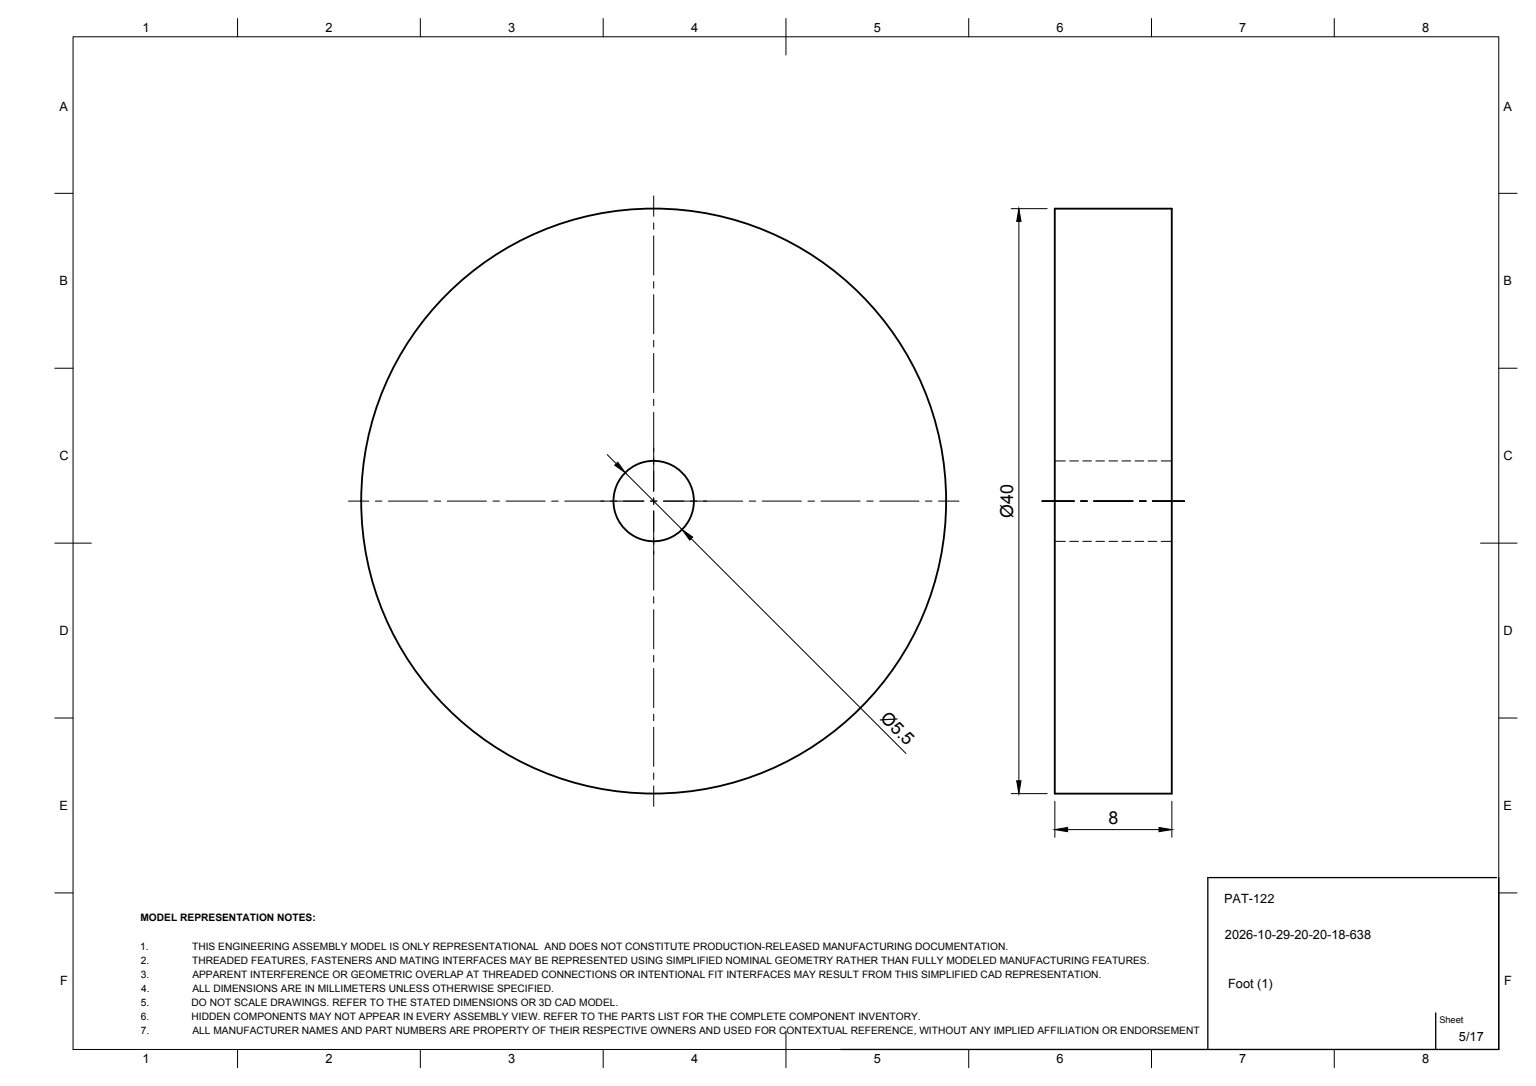
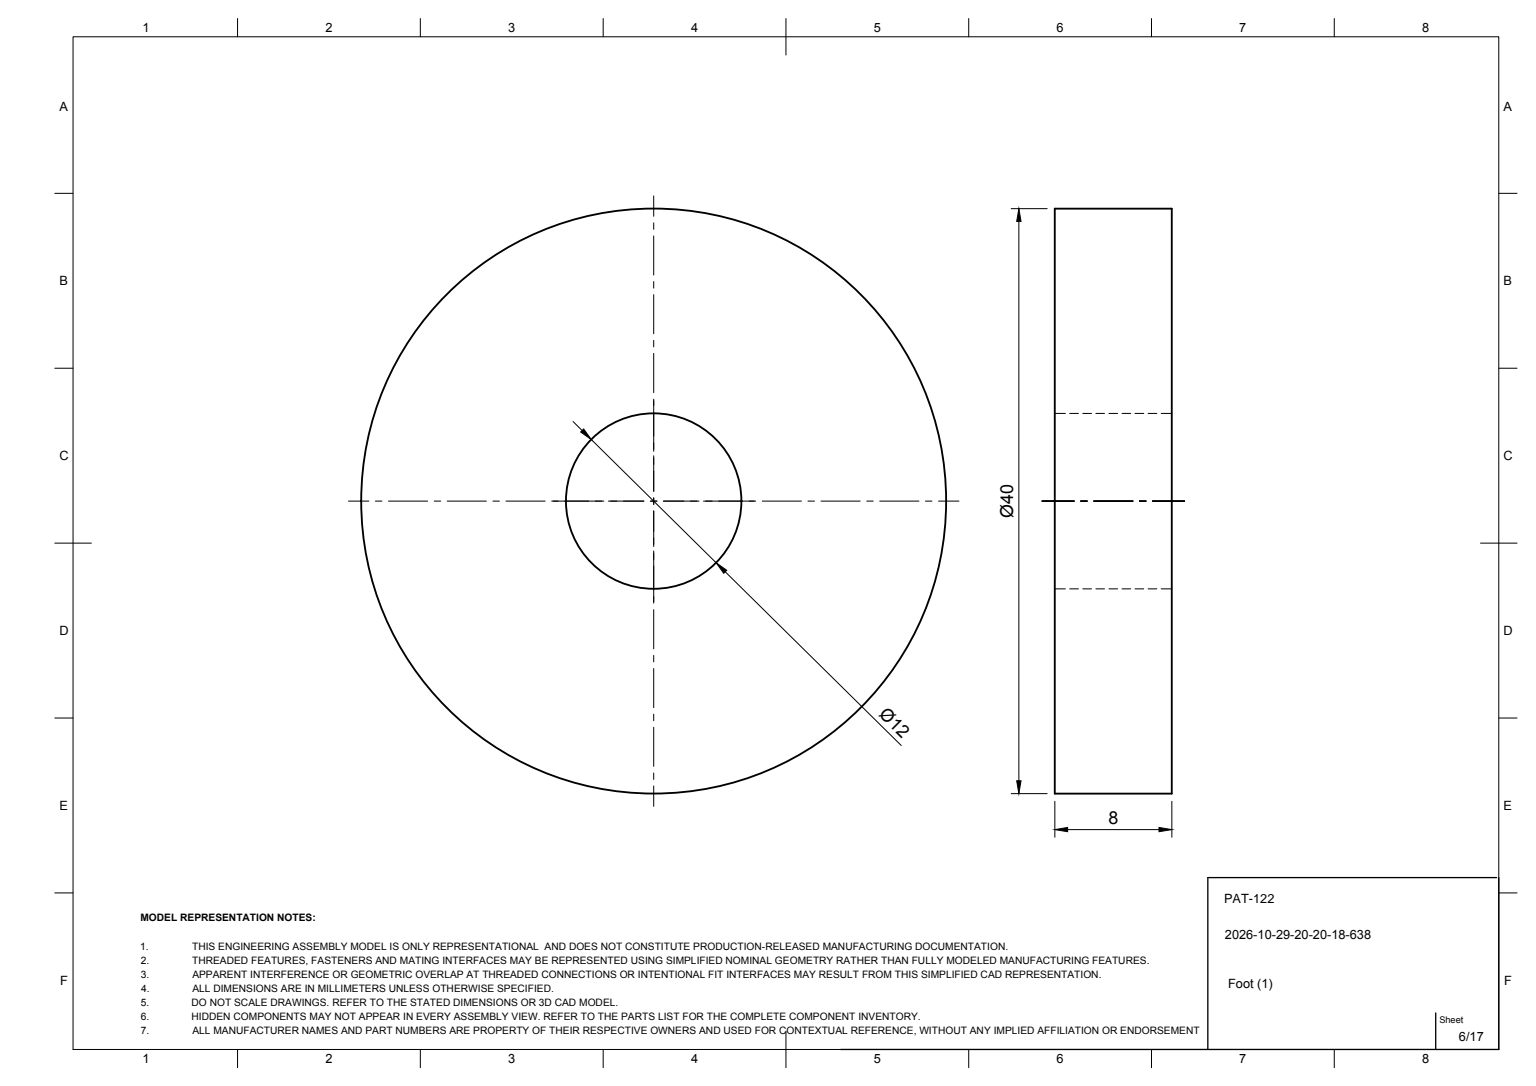
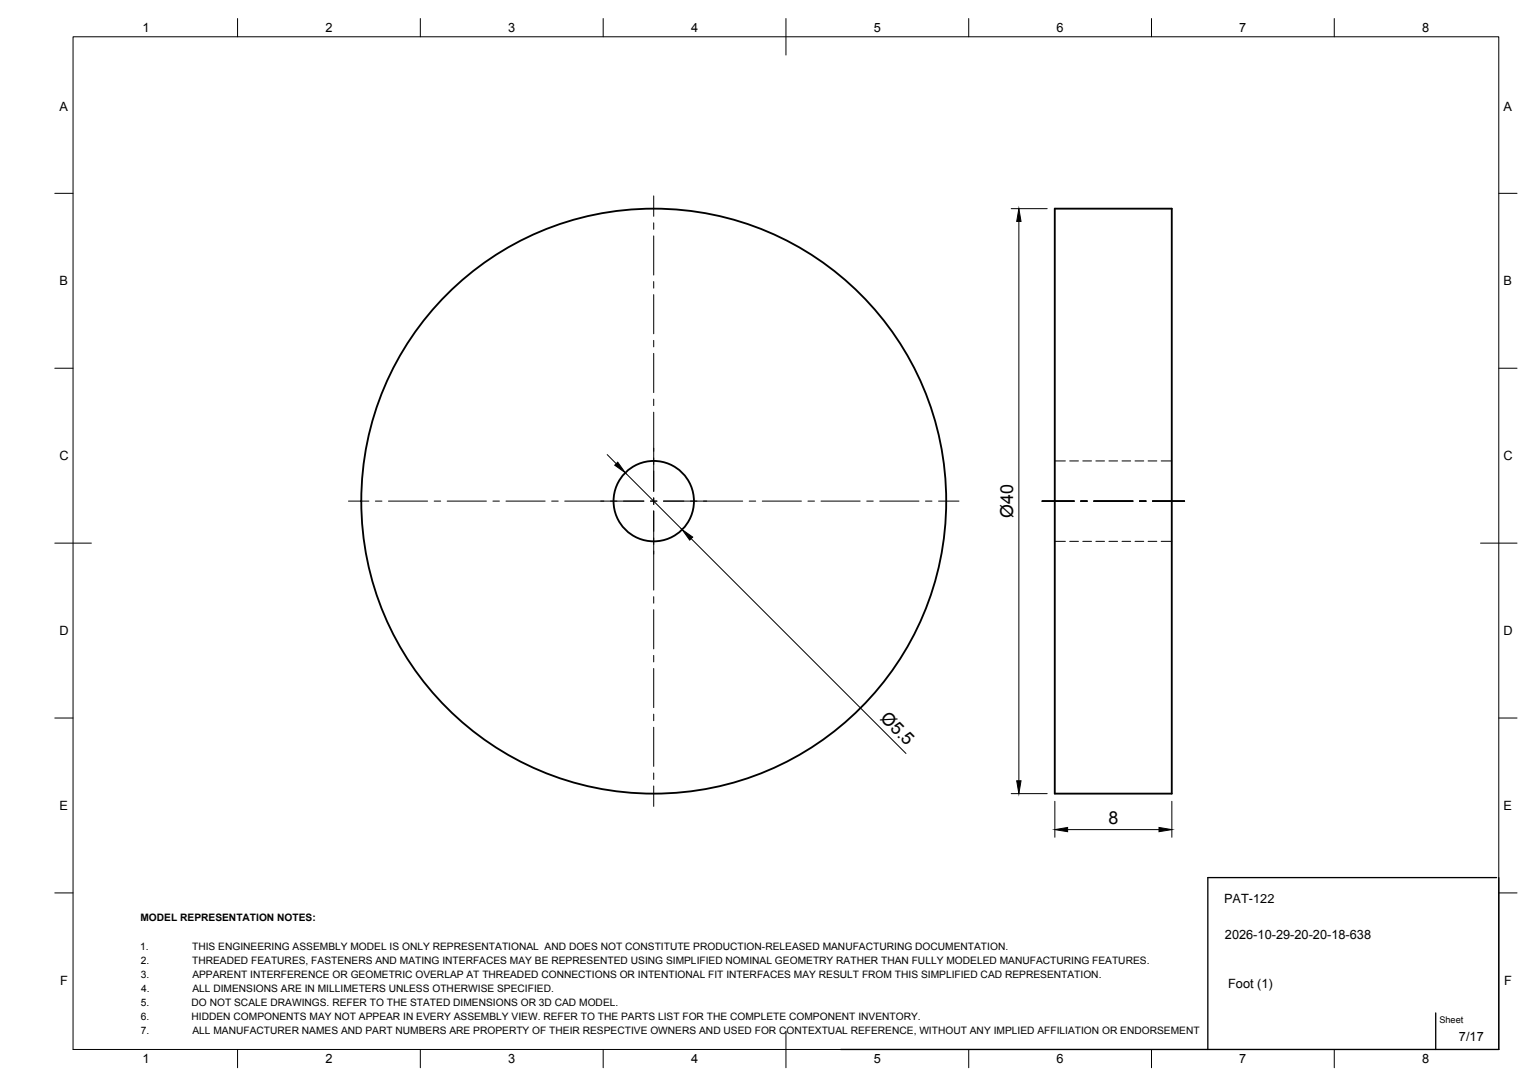
ISO-10303-21;
HEADER;
/* Generated by software containing ST-Developer
 * from STEP Tools, Inc. (www.steptools.com) 
 */

FILE_DESCRIPTION(
/* description */ ('PAT-122'),
/* implementation_level */ '2;1');

FILE_NAME(
/* name */ 'Foot (1).step',
/* time_stamp */ '2026-10-29T20:20:12-07:00',
/* author */ (''),
/* organization */ (''),
/* preprocessor_version */ 'ST-DEVELOPER v20.2',
/* originating_system */ 'Autodesk Translation Framework v15.17.0.0',
/* authorisation */ '');

FILE_SCHEMA (('AUTOMOTIVE_DESIGN { 1 0 10303 214 3 1 1 }'));
ENDSEC;

DATA;
#10=MECHANICAL_DESIGN_GEOMETRIC_PRESENTATION_REPRESENTATION('',(#493),#10019);
#449=SHAPE_REPRESENTATION_RELATIONSHIP('SRR','None',#10170,#471);
#471=ADVANCED_BREP_SHAPE_REPRESENTATION('',(#515),#9999);
#493=STYLED_ITEM('',(#10362),#515);
#515=MANIFOLD_SOLID_BREP('Body1',#5615);
#535=FACE_BOUND('',#1132,.T.);
#536=FACE_BOUND('',#1134,.T.);
#613=PLANE('',#5908);
#614=PLANE('',#5909);
#833=FACE_OUTER_BOUND('',#1129,.T.);
#834=FACE_OUTER_BOUND('',#1130,.T.);
#835=FACE_OUTER_BOUND('',#1131,.T.);
#836=FACE_OUTER_BOUND('',#1133,.T.);
#1129=EDGE_LOOP('',(#3889,#3890,#3891,#3892));
#1130=EDGE_LOOP('',(#3893,#3894,#3895,#3896));
#1131=EDGE_LOOP('',(#3897));
#1132=EDGE_LOOP('',(#3898));
#1133=EDGE_LOOP('',(#3899));
#1134=EDGE_LOOP('',(#3900));
#1491=LINE('',#8094,#2035);
#1492=LINE('',#8100,#2036);
#2035=VECTOR('',#6474,0.274999999999999);
#2036=VECTOR('',#6481,2.);
#2583=CIRCLE('',#5903,0.274999999999999);
#2584=CIRCLE('',#5904,0.274999999999999);
#2585=CIRCLE('',#5906,2.);
#2586=CIRCLE('',#5907,2.);
#2713=VERTEX_POINT('',#8091);
#2714=VERTEX_POINT('',#8093);
#2715=VERTEX_POINT('',#8097);
#2716=VERTEX_POINT('',#8099);
#3179=EDGE_CURVE('',#2713,#2713,#2583,.T.);
#3180=EDGE_CURVE('',#2713,#2714,#1491,.T.);
#3181=EDGE_CURVE('',#2714,#2714,#2584,.T.);
#3182=EDGE_CURVE('',#2715,#2715,#2585,.T.);
#3183=EDGE_CURVE('',#2715,#2716,#1492,.T.);
#3184=EDGE_CURVE('',#2716,#2716,#2586,.T.);
#3889=ORIENTED_EDGE('',*,*,#3179,.F.);
#3890=ORIENTED_EDGE('',*,*,#3180,.T.);
#3891=ORIENTED_EDGE('',*,*,#3181,.T.);
#3892=ORIENTED_EDGE('',*,*,#3180,.F.);
#3893=ORIENTED_EDGE('',*,*,#3182,.F.);
#3894=ORIENTED_EDGE('',*,*,#3183,.T.);
#3895=ORIENTED_EDGE('',*,*,#3184,.T.);
#3896=ORIENTED_EDGE('',*,*,#3183,.F.);
#3897=ORIENTED_EDGE('',*,*,#3182,.T.);
#3898=ORIENTED_EDGE('',*,*,#3179,.T.);
#3899=ORIENTED_EDGE('',*,*,#3184,.F.);
#3900=ORIENTED_EDGE('',*,*,#3181,.F.);
#5265=CYLINDRICAL_SURFACE('',#5902,0.274999999999999);
#5266=CYLINDRICAL_SURFACE('',#5905,2.);
#5329=ADVANCED_FACE('',(#833),#5265,.F.);
#5330=ADVANCED_FACE('',(#834),#5266,.T.);
#5331=ADVANCED_FACE('',(#835,#535),#613,.T.);
#5332=ADVANCED_FACE('',(#836,#536),#614,.F.);
#5615=CLOSED_SHELL('',(#5329,#5330,#5331,#5332));
#5901=AXIS2_PLACEMENT_3D('',#8089,#6468,#6469);
#5902=AXIS2_PLACEMENT_3D('',#8090,#6470,#6471);
#5903=AXIS2_PLACEMENT_3D('',#8092,#6472,#6473);
#5904=AXIS2_PLACEMENT_3D('',#8095,#6475,#6476);
#5905=AXIS2_PLACEMENT_3D('',#8096,#6477,#6478);
#5906=AXIS2_PLACEMENT_3D('',#8098,#6479,#6480);
#5907=AXIS2_PLACEMENT_3D('',#8101,#6482,#6483);
#5908=AXIS2_PLACEMENT_3D('',#8102,#6484,#6485);
#5909=AXIS2_PLACEMENT_3D('',#8103,#6486,#6487);
#6468=DIRECTION('axis',(0.,0.,1.));
#6469=DIRECTION('refdir',(1.,0.,0.));
#6470=DIRECTION('center_axis',(0.,0.,1.));
#6471=DIRECTION('ref_axis',(1.,0.,0.));
#6472=DIRECTION('center_axis',(0.,0.,-1.));
#6473=DIRECTION('ref_axis',(1.,0.,0.));
#6474=DIRECTION('',(0.,0.,-1.));
#6475=DIRECTION('center_axis',(0.,0.,-1.));
#6476=DIRECTION('ref_axis',(1.,0.,0.));
#6477=DIRECTION('center_axis',(0.,0.,1.));
#6478=DIRECTION('ref_axis',(1.,0.,0.));
#6479=DIRECTION('center_axis',(0.,0.,1.));
#6480=DIRECTION('ref_axis',(1.,0.,0.));
#6481=DIRECTION('',(0.,0.,-1.));
#6482=DIRECTION('center_axis',(0.,0.,1.));
#6483=DIRECTION('ref_axis',(1.,0.,0.));
#6484=DIRECTION('center_axis',(0.,0.,1.));
#6485=DIRECTION('ref_axis',(1.,0.,0.));
#6486=DIRECTION('center_axis',(0.,0.,1.));
#6487=DIRECTION('ref_axis',(1.,0.,0.));
#8089=CARTESIAN_POINT('',(0.,0.,0.));
#8090=CARTESIAN_POINT('Origin',(-19.,19.,-0.8));
#8091=CARTESIAN_POINT('',(-19.275,19.,0.));
#8092=CARTESIAN_POINT('Origin',(-19.,19.,0.));
#8093=CARTESIAN_POINT('',(-19.275,19.,-0.8));
#8094=CARTESIAN_POINT('',(-19.275,19.,-0.8));
#8095=CARTESIAN_POINT('Origin',(-19.,19.,-0.8));
#8096=CARTESIAN_POINT('Origin',(-19.,19.,-0.8));
#8097=CARTESIAN_POINT('',(-21.,19.,0.));
#8098=CARTESIAN_POINT('Origin',(-19.,19.,0.));
#8099=CARTESIAN_POINT('',(-21.,19.,-0.8));
#8100=CARTESIAN_POINT('',(-21.,19.,-0.8));
#8101=CARTESIAN_POINT('Origin',(-19.,19.,-0.8));
#8102=CARTESIAN_POINT('Origin',(-19.,19.,0.));
#8103=CARTESIAN_POINT('Origin',(-19.,19.,-0.8));
#9975=UNCERTAINTY_MEASURE_WITH_UNIT(LENGTH_MEASURE(0.001),#10020,
'DISTANCE_ACCURACY_VALUE',
'Maximum model space distance between geometric entities at asserted c
onnectivities');
#9995=UNCERTAINTY_MEASURE_WITH_UNIT(LENGTH_MEASURE(0.001),#10020,
'DISTANCE_ACCURACY_VALUE',
'Maximum model space distance between geometric entities at asserted c
onnectivities');
#9999=(
GEOMETRIC_REPRESENTATION_CONTEXT(3)
GLOBAL_UNCERTAINTY_ASSIGNED_CONTEXT((#9975))
GLOBAL_UNIT_ASSIGNED_CONTEXT((#10020,#10022,#10023))
REPRESENTATION_CONTEXT('','3D')
);
#10019=(
GEOMETRIC_REPRESENTATION_CONTEXT(3)
GLOBAL_UNCERTAINTY_ASSIGNED_CONTEXT((#9995))
GLOBAL_UNIT_ASSIGNED_CONTEXT((#10020,#10022,#10023))
REPRESENTATION_CONTEXT('','3D')
);
#10020=(
LENGTH_UNIT()
NAMED_UNIT(*)
SI_UNIT(.CENTI.,.METRE.)
);
#10022=(
NAMED_UNIT(*)
PLANE_ANGLE_UNIT()
SI_UNIT($,.RADIAN.)
);
#10023=(
NAMED_UNIT(*)
SI_UNIT($,.STERADIAN.)
SOLID_ANGLE_UNIT()
);
#10027=SHAPE_DEFINITION_REPRESENTATION(#10050,#10170);
#10050=PRODUCT_DEFINITION_SHAPE('',$,#10194);
#10170=SHAPE_REPRESENTATION('',(#5901),#9999);
#10190=PRODUCT_DEFINITION_CONTEXT('part definition',#10261,'design');
#10194=PRODUCT_DEFINITION('Foot (1)','Foot (1)',#10217,#10190);
#10217=PRODUCT_DEFINITION_FORMATION('',$,#10266);
#10261=APPLICATION_CONTEXT(
'Core Data for Automotive Mechanical Design Process');
#10262=PRODUCT_CONTEXT('part definition',#10261,'mechanical');
#10266=PRODUCT('Foot (1)','Foot (1)','Foot (1)',(#10262));
#10356=COLOUR_RGB('Off White',0.89,0.88,0.83);
#10357=FILL_AREA_STYLE_COLOUR('',#10356);
#10358=FILL_AREA_STYLE('',(#10357));
#10359=SURFACE_STYLE_FILL_AREA(#10358);
#10360=SURFACE_SIDE_STYLE('',(#10359));
#10361=SURFACE_STYLE_USAGE(.BOTH.,#10360);
#10362=PRESENTATION_STYLE_ASSIGNMENT((#10361));
ENDSEC;
END-ISO-10303-21;
